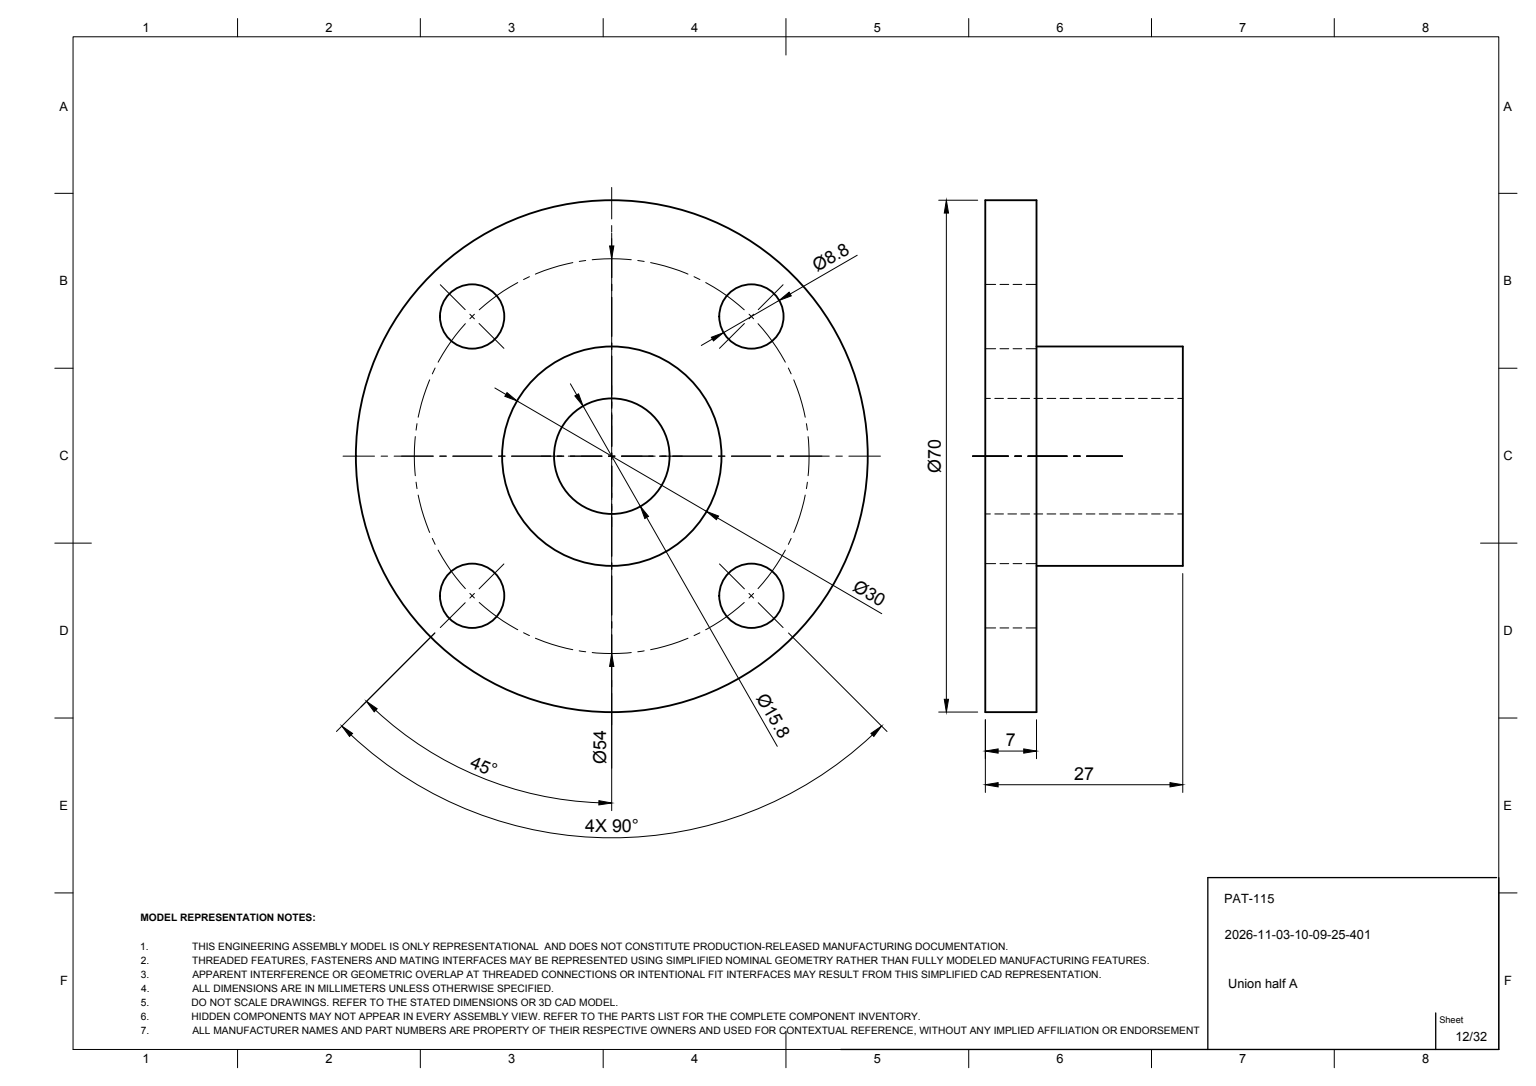
ISO-10303-21;
HEADER;
/* Generated by software containing ST-Developer
 * from STEP Tools, Inc. (www.steptools.com) 
 */

FILE_DESCRIPTION(
/* description */ ('Union bypass pipe loop'),
/* implementation_level */ '2;1');

FILE_NAME(
/* name */ 'Union half A.step',
/* time_stamp */ '2026-10-27T21:00:29-07:00',
/* author */ (''),
/* organization */ (''),
/* preprocessor_version */ 'ST-DEVELOPER v20.2',
/* originating_system */ 'Autodesk Translation Framework v15.17.0.0',
/* authorisation */ '');

FILE_SCHEMA (('AUTOMOTIVE_DESIGN { 1 0 10303 214 3 1 1 }'));
ENDSEC;

DATA;
#10=MECHANICAL_DESIGN_GEOMETRIC_PRESENTATION_REPRESENTATION('',(#466),#10095);
#402=SHAPE_REPRESENTATION_RELATIONSHIP('SRR','None',#10271,#434);
#434=ADVANCED_BREP_SHAPE_REPRESENTATION('',(#496),#10083);
#466=STYLED_ITEM('',(#10514),#496);
#496=MANIFOLD_SOLID_BREP('Body1',#5539);
#599=FACE_BOUND('',#1475,.T.);
#600=FACE_BOUND('',#1476,.T.);
#601=FACE_BOUND('',#1477,.T.);
#602=FACE_BOUND('',#1478,.T.);
#603=FACE_BOUND('',#1479,.T.);
#604=FACE_BOUND('',#1484,.T.);
#605=FACE_BOUND('',#1485,.T.);
#606=FACE_BOUND('',#1486,.T.);
#607=FACE_BOUND('',#1487,.T.);
#608=FACE_BOUND('',#1488,.T.);
#609=FACE_BOUND('',#1490,.T.);
#754=PLANE('',#6388);
#755=PLANE('',#6398);
#756=PLANE('',#6399);
#1050=FACE_OUTER_BOUND('',#1470,.T.);
#1051=FACE_OUTER_BOUND('',#1471,.T.);
#1052=FACE_OUTER_BOUND('',#1472,.T.);
#1053=FACE_OUTER_BOUND('',#1473,.T.);
#1054=FACE_OUTER_BOUND('',#1474,.T.);
#1055=FACE_OUTER_BOUND('',#1480,.T.);
#1056=FACE_OUTER_BOUND('',#1481,.T.);
#1057=FACE_OUTER_BOUND('',#1482,.T.);
#1058=FACE_OUTER_BOUND('',#1483,.T.);
#1059=FACE_OUTER_BOUND('',#1489,.T.);
#1470=EDGE_LOOP('',(#4600,#4601,#4602,#4603));
#1471=EDGE_LOOP('',(#4604,#4605,#4606,#4607));
#1472=EDGE_LOOP('',(#4608,#4609,#4610,#4611));
#1473=EDGE_LOOP('',(#4612,#4613,#4614,#4615));
#1474=EDGE_LOOP('',(#4616));
#1475=EDGE_LOOP('',(#4617));
#1476=EDGE_LOOP('',(#4618));
#1477=EDGE_LOOP('',(#4619));
#1478=EDGE_LOOP('',(#4620));
#1479=EDGE_LOOP('',(#4621));
#1480=EDGE_LOOP('',(#4622,#4623,#4624,#4625));
#1481=EDGE_LOOP('',(#4626,#4627,#4628,#4629));
#1482=EDGE_LOOP('',(#4630,#4631,#4632,#4633));
#1483=EDGE_LOOP('',(#4634));
#1484=EDGE_LOOP('',(#4635));
#1485=EDGE_LOOP('',(#4636));
#1486=EDGE_LOOP('',(#4637));
#1487=EDGE_LOOP('',(#4638));
#1488=EDGE_LOOP('',(#4639));
#1489=EDGE_LOOP('',(#4640));
#1490=EDGE_LOOP('',(#4641));
#1846=LINE('',#9439,#2222);
#1847=LINE('',#9445,#2223);
#1848=LINE('',#9451,#2224);
#1849=LINE('',#9457,#2225);
#1850=LINE('',#9467,#2226);
#1851=LINE('',#9472,#2227);
#1852=LINE('',#9476,#2228);
#2222=VECTOR('',#7788,0.44);
#2223=VECTOR('',#7795,0.44);
#2224=VECTOR('',#7802,0.44);
#2225=VECTOR('',#7809,0.44);
#2226=VECTOR('',#7822,3.5);
#2227=VECTOR('',#7827,0.79);
#2228=VECTOR('',#7832,1.5);
#2555=CIRCLE('',#6377,0.44);
#2556=CIRCLE('',#6378,0.44);
#2557=CIRCLE('',#6380,0.44);
#2558=CIRCLE('',#6381,0.44);
#2559=CIRCLE('',#6383,0.44);
#2560=CIRCLE('',#6384,0.44);
#2561=CIRCLE('',#6386,0.44);
#2562=CIRCLE('',#6387,0.44);
#2563=CIRCLE('',#6389,3.5);
#2564=CIRCLE('',#6390,1.5);
#2565=CIRCLE('',#6392,3.5);
#2566=CIRCLE('',#6394,0.79);
#2567=CIRCLE('',#6395,0.79);
#2568=CIRCLE('',#6397,1.5);
#2912=VERTEX_POINT('',#9436);
#2913=VERTEX_POINT('',#9438);
#2914=VERTEX_POINT('',#9442);
#2915=VERTEX_POINT('',#9444);
#2916=VERTEX_POINT('',#9448);
#2917=VERTEX_POINT('',#9450);
#2918=VERTEX_POINT('',#9454);
#2919=VERTEX_POINT('',#9456);
#2920=VERTEX_POINT('',#9460);
#2921=VERTEX_POINT('',#9462);
#2922=VERTEX_POINT('',#9465);
#2923=VERTEX_POINT('',#9469);
#2924=VERTEX_POINT('',#9471);
#2925=VERTEX_POINT('',#9475);
#3498=EDGE_CURVE('',#2912,#2912,#2555,.T.);
#3499=EDGE_CURVE('',#2912,#2913,#1846,.T.);
#3500=EDGE_CURVE('',#2913,#2913,#2556,.T.);
#3501=EDGE_CURVE('',#2914,#2914,#2557,.T.);
#3502=EDGE_CURVE('',#2914,#2915,#1847,.T.);
#3503=EDGE_CURVE('',#2915,#2915,#2558,.T.);
#3504=EDGE_CURVE('',#2916,#2916,#2559,.T.);
#3505=EDGE_CURVE('',#2916,#2917,#1848,.T.);
#3506=EDGE_CURVE('',#2917,#2917,#2560,.T.);
#3507=EDGE_CURVE('',#2918,#2918,#2561,.T.);
#3508=EDGE_CURVE('',#2918,#2919,#1849,.T.);
#3509=EDGE_CURVE('',#2919,#2919,#2562,.T.);
#3510=EDGE_CURVE('',#2920,#2920,#2563,.T.);
#3511=EDGE_CURVE('',#2921,#2921,#2564,.T.);
#3512=EDGE_CURVE('',#2922,#2922,#2565,.T.);
#3513=EDGE_CURVE('',#2922,#2920,#1850,.T.);
#3514=EDGE_CURVE('',#2923,#2923,#2566,.T.);
#3515=EDGE_CURVE('',#2923,#2924,#1851,.T.);
#3516=EDGE_CURVE('',#2924,#2924,#2567,.T.);
#3517=EDGE_CURVE('',#2921,#2925,#1852,.T.);
#3518=EDGE_CURVE('',#2925,#2925,#2568,.T.);
#4600=ORIENTED_EDGE('',*,*,#3498,.F.);
#4601=ORIENTED_EDGE('',*,*,#3499,.T.);
#4602=ORIENTED_EDGE('',*,*,#3500,.F.);
#4603=ORIENTED_EDGE('',*,*,#3499,.F.);
#4604=ORIENTED_EDGE('',*,*,#3501,.F.);
#4605=ORIENTED_EDGE('',*,*,#3502,.T.);
#4606=ORIENTED_EDGE('',*,*,#3503,.F.);
#4607=ORIENTED_EDGE('',*,*,#3502,.F.);
#4608=ORIENTED_EDGE('',*,*,#3504,.F.);
#4609=ORIENTED_EDGE('',*,*,#3505,.T.);
#4610=ORIENTED_EDGE('',*,*,#3506,.F.);
#4611=ORIENTED_EDGE('',*,*,#3505,.F.);
#4612=ORIENTED_EDGE('',*,*,#3507,.F.);
#4613=ORIENTED_EDGE('',*,*,#3508,.T.);
#4614=ORIENTED_EDGE('',*,*,#3509,.F.);
#4615=ORIENTED_EDGE('',*,*,#3508,.F.);
#4616=ORIENTED_EDGE('',*,*,#3510,.F.);
#4617=ORIENTED_EDGE('',*,*,#3511,.F.);
#4618=ORIENTED_EDGE('',*,*,#3507,.T.);
#4619=ORIENTED_EDGE('',*,*,#3504,.T.);
#4620=ORIENTED_EDGE('',*,*,#3501,.T.);
#4621=ORIENTED_EDGE('',*,*,#3498,.T.);
#4622=ORIENTED_EDGE('',*,*,#3512,.F.);
#4623=ORIENTED_EDGE('',*,*,#3513,.T.);
#4624=ORIENTED_EDGE('',*,*,#3510,.T.);
#4625=ORIENTED_EDGE('',*,*,#3513,.F.);
#4626=ORIENTED_EDGE('',*,*,#3514,.F.);
#4627=ORIENTED_EDGE('',*,*,#3515,.T.);
#4628=ORIENTED_EDGE('',*,*,#3516,.T.);
#4629=ORIENTED_EDGE('',*,*,#3515,.F.);
#4630=ORIENTED_EDGE('',*,*,#3511,.T.);
#4631=ORIENTED_EDGE('',*,*,#3517,.T.);
#4632=ORIENTED_EDGE('',*,*,#3518,.T.);
#4633=ORIENTED_EDGE('',*,*,#3517,.F.);
#4634=ORIENTED_EDGE('',*,*,#3512,.T.);
#4635=ORIENTED_EDGE('',*,*,#3514,.T.);
#4636=ORIENTED_EDGE('',*,*,#3509,.T.);
#4637=ORIENTED_EDGE('',*,*,#3506,.T.);
#4638=ORIENTED_EDGE('',*,*,#3503,.T.);
#4639=ORIENTED_EDGE('',*,*,#3500,.T.);
#4640=ORIENTED_EDGE('',*,*,#3518,.F.);
#4641=ORIENTED_EDGE('',*,*,#3516,.F.);
#5158=CYLINDRICAL_SURFACE('',#6376,0.44);
#5159=CYLINDRICAL_SURFACE('',#6379,0.44);
#5160=CYLINDRICAL_SURFACE('',#6382,0.44);
#5161=CYLINDRICAL_SURFACE('',#6385,0.44);
#5162=CYLINDRICAL_SURFACE('',#6391,3.5);
#5163=CYLINDRICAL_SURFACE('',#6393,0.79);
#5164=CYLINDRICAL_SURFACE('',#6396,1.5);
#5399=ADVANCED_FACE('',(#1050),#5158,.F.);
#5400=ADVANCED_FACE('',(#1051),#5159,.F.);
#5401=ADVANCED_FACE('',(#1052),#5160,.F.);
#5402=ADVANCED_FACE('',(#1053),#5161,.F.);
#5403=ADVANCED_FACE('',(#1054,#599,#600,#601,#602,#603),#754,.F.);
#5404=ADVANCED_FACE('',(#1055),#5162,.T.);
#5405=ADVANCED_FACE('',(#1056),#5163,.F.);
#5406=ADVANCED_FACE('',(#1057),#5164,.T.);
#5407=ADVANCED_FACE('',(#1058,#604,#605,#606,#607,#608),#755,.T.);
#5408=ADVANCED_FACE('',(#1059,#609),#756,.F.);
#5539=CLOSED_SHELL('',(#5399,#5400,#5401,#5402,#5403,#5404,#5405,#5406,
#5407,#5408));
#6375=AXIS2_PLACEMENT_3D('',#9434,#7782,#7783);
#6376=AXIS2_PLACEMENT_3D('',#9435,#7784,#7785);
#6377=AXIS2_PLACEMENT_3D('',#9437,#7786,#7787);
#6378=AXIS2_PLACEMENT_3D('',#9440,#7789,#7790);
#6379=AXIS2_PLACEMENT_3D('',#9441,#7791,#7792);
#6380=AXIS2_PLACEMENT_3D('',#9443,#7793,#7794);
#6381=AXIS2_PLACEMENT_3D('',#9446,#7796,#7797);
#6382=AXIS2_PLACEMENT_3D('',#9447,#7798,#7799);
#6383=AXIS2_PLACEMENT_3D('',#9449,#7800,#7801);
#6384=AXIS2_PLACEMENT_3D('',#9452,#7803,#7804);
#6385=AXIS2_PLACEMENT_3D('',#9453,#7805,#7806);
#6386=AXIS2_PLACEMENT_3D('',#9455,#7807,#7808);
#6387=AXIS2_PLACEMENT_3D('',#9458,#7810,#7811);
#6388=AXIS2_PLACEMENT_3D('',#9459,#7812,#7813);
#6389=AXIS2_PLACEMENT_3D('',#9461,#7814,#7815);
#6390=AXIS2_PLACEMENT_3D('',#9463,#7816,#7817);
#6391=AXIS2_PLACEMENT_3D('',#9464,#7818,#7819);
#6392=AXIS2_PLACEMENT_3D('',#9466,#7820,#7821);
#6393=AXIS2_PLACEMENT_3D('',#9468,#7823,#7824);
#6394=AXIS2_PLACEMENT_3D('',#9470,#7825,#7826);
#6395=AXIS2_PLACEMENT_3D('',#9473,#7828,#7829);
#6396=AXIS2_PLACEMENT_3D('',#9474,#7830,#7831);
#6397=AXIS2_PLACEMENT_3D('',#9477,#7833,#7834);
#6398=AXIS2_PLACEMENT_3D('',#9478,#7835,#7836);
#6399=AXIS2_PLACEMENT_3D('',#9479,#7837,#7838);
#7782=DIRECTION('axis',(0.,0.,1.));
#7783=DIRECTION('refdir',(1.,0.,0.));
#7784=DIRECTION('center_axis',(1.,0.,0.));
#7785=DIRECTION('ref_axis',(0.,0.,-1.));
#7786=DIRECTION('center_axis',(1.,0.,0.));
#7787=DIRECTION('ref_axis',(0.,0.,-1.));
#7788=DIRECTION('',(1.,0.,0.));
#7789=DIRECTION('center_axis',(-1.,0.,0.));
#7790=DIRECTION('ref_axis',(0.,0.,-1.));
#7791=DIRECTION('center_axis',(1.,0.,0.));
#7792=DIRECTION('ref_axis',(0.,0.,-1.));
#7793=DIRECTION('center_axis',(1.,0.,0.));
#7794=DIRECTION('ref_axis',(0.,0.,-1.));
#7795=DIRECTION('',(1.,0.,0.));
#7796=DIRECTION('center_axis',(-1.,0.,0.));
#7797=DIRECTION('ref_axis',(0.,0.,-1.));
#7798=DIRECTION('center_axis',(1.,0.,0.));
#7799=DIRECTION('ref_axis',(0.,0.,-1.));
#7800=DIRECTION('center_axis',(1.,0.,0.));
#7801=DIRECTION('ref_axis',(0.,0.,-1.));
#7802=DIRECTION('',(1.,0.,0.));
#7803=DIRECTION('center_axis',(-1.,0.,0.));
#7804=DIRECTION('ref_axis',(0.,0.,-1.));
#7805=DIRECTION('center_axis',(1.,0.,0.));
#7806=DIRECTION('ref_axis',(0.,0.,-1.));
#7807=DIRECTION('center_axis',(1.,0.,0.));
#7808=DIRECTION('ref_axis',(0.,0.,-1.));
#7809=DIRECTION('',(1.,0.,0.));
#7810=DIRECTION('center_axis',(-1.,0.,0.));
#7811=DIRECTION('ref_axis',(0.,0.,-1.));
#7812=DIRECTION('center_axis',(1.,0.,0.));
#7813=DIRECTION('ref_axis',(0.,0.,-1.));
#7814=DIRECTION('center_axis',(1.,0.,0.));
#7815=DIRECTION('ref_axis',(0.,0.,-1.));
#7816=DIRECTION('center_axis',(-1.,0.,0.));
#7817=DIRECTION('ref_axis',(0.,0.,-1.));
#7818=DIRECTION('center_axis',(1.,0.,0.));
#7819=DIRECTION('ref_axis',(0.,0.,-1.));
#7820=DIRECTION('center_axis',(1.,0.,0.));
#7821=DIRECTION('ref_axis',(0.,0.,-1.));
#7822=DIRECTION('',(-1.,0.,0.));
#7823=DIRECTION('center_axis',(1.,0.,0.));
#7824=DIRECTION('ref_axis',(0.,0.,-1.));
#7825=DIRECTION('center_axis',(-1.,0.,0.));
#7826=DIRECTION('ref_axis',(0.,0.,-1.));
#7827=DIRECTION('',(-1.,0.,0.));
#7828=DIRECTION('center_axis',(-1.,0.,0.));
#7829=DIRECTION('ref_axis',(0.,0.,-1.));
#7830=DIRECTION('center_axis',(1.,0.,0.));
#7831=DIRECTION('ref_axis',(0.,0.,-1.));
#7832=DIRECTION('',(-1.,0.,0.));
#7833=DIRECTION('center_axis',(1.,0.,0.));
#7834=DIRECTION('ref_axis',(0.,0.,-1.));
#7835=DIRECTION('center_axis',(1.,0.,0.));
#7836=DIRECTION('ref_axis',(0.,0.,-1.));
#7837=DIRECTION('center_axis',(1.,0.,0.));
#7838=DIRECTION('ref_axis',(0.,0.,-1.));
#9434=CARTESIAN_POINT('',(0.,0.,0.));
#9435=CARTESIAN_POINT('Origin',(-0.9,-1.90918830920368,4.09081169079632));
#9436=CARTESIAN_POINT('',(-0.8,-1.90918830920368,4.53081169079632));
#9437=CARTESIAN_POINT('Origin',(-0.8,-1.90918830920368,4.09081169079632));
#9438=CARTESIAN_POINT('',(-0.1,-1.90918830920368,4.53081169079632));
#9439=CARTESIAN_POINT('',(-0.9,-1.90918830920368,4.53081169079632));
#9440=CARTESIAN_POINT('Origin',(-0.1,-1.90918830920368,4.09081169079632));
#9441=CARTESIAN_POINT('Origin',(-0.9,-1.90918830920368,7.90918830920368));
#9442=CARTESIAN_POINT('',(-0.8,-1.90918830920368,8.34918830920368));
#9443=CARTESIAN_POINT('Origin',(-0.8,-1.90918830920368,7.90918830920368));
#9444=CARTESIAN_POINT('',(-0.1,-1.90918830920368,8.34918830920368));
#9445=CARTESIAN_POINT('',(-0.9,-1.90918830920368,8.34918830920368));
#9446=CARTESIAN_POINT('Origin',(-0.1,-1.90918830920368,7.90918830920368));
#9447=CARTESIAN_POINT('Origin',(-0.9,1.90918830920368,7.90918830920368));
#9448=CARTESIAN_POINT('',(-0.8,1.90918830920368,8.34918830920368));
#9449=CARTESIAN_POINT('Origin',(-0.8,1.90918830920368,7.90918830920368));
#9450=CARTESIAN_POINT('',(-0.1,1.90918830920368,8.34918830920368));
#9451=CARTESIAN_POINT('',(-0.9,1.90918830920368,8.34918830920368));
#9452=CARTESIAN_POINT('Origin',(-0.1,1.90918830920368,7.90918830920368));
#9453=CARTESIAN_POINT('Origin',(-0.9,1.90918830920368,4.09081169079632));
#9454=CARTESIAN_POINT('',(-0.8,1.90918830920368,4.53081169079632));
#9455=CARTESIAN_POINT('Origin',(-0.8,1.90918830920368,4.09081169079632));
#9456=CARTESIAN_POINT('',(-0.1,1.90918830920368,4.53081169079632));
#9457=CARTESIAN_POINT('',(-0.9,1.90918830920368,4.53081169079632));
#9458=CARTESIAN_POINT('Origin',(-0.1,1.90918830920368,4.09081169079632));
#9459=CARTESIAN_POINT('Origin',(-0.8,0.,6.));
#9460=CARTESIAN_POINT('',(-0.8,-4.28626379701574E-16,9.5));
#9461=CARTESIAN_POINT('Origin',(-0.8,0.,6.));
#9462=CARTESIAN_POINT('',(-0.8,1.83697019872103E-16,7.5));
#9463=CARTESIAN_POINT('Origin',(-0.8,0.,6.));
#9464=CARTESIAN_POINT('Origin',(-0.8,0.,6.));
#9465=CARTESIAN_POINT('',(-0.1,-4.28626379701574E-16,9.5));
#9466=CARTESIAN_POINT('Origin',(-0.1,0.,6.));
#9467=CARTESIAN_POINT('',(-0.8,-4.28626379701574E-16,9.5));
#9468=CARTESIAN_POINT('Origin',(-2.8,0.,6.));
#9469=CARTESIAN_POINT('',(-0.1,-9.67470971326409E-17,6.79));
#9470=CARTESIAN_POINT('Origin',(-0.1,0.,6.));
#9471=CARTESIAN_POINT('',(-2.8,-9.67470971326409E-17,6.79));
#9472=CARTESIAN_POINT('',(-2.8,-9.67470971326409E-17,6.79));
#9473=CARTESIAN_POINT('Origin',(-2.8,0.,6.));
#9474=CARTESIAN_POINT('Origin',(-2.8,0.,6.));
#9475=CARTESIAN_POINT('',(-2.8,-1.83697019872103E-16,7.5));
#9476=CARTESIAN_POINT('',(-2.8,-1.83697019872103E-16,7.5));
#9477=CARTESIAN_POINT('Origin',(-2.8,0.,6.));
#9478=CARTESIAN_POINT('Origin',(-0.1,0.,6.));
#9479=CARTESIAN_POINT('Origin',(-2.8,0.,6.));
#10046=UNCERTAINTY_MEASURE_WITH_UNIT(LENGTH_MEASURE(0.001),#10096,
'DISTANCE_ACCURACY_VALUE',
'Maximum model space distance between geometric entities at asserted c
onnectivities');
#10058=UNCERTAINTY_MEASURE_WITH_UNIT(LENGTH_MEASURE(0.001),#10096,
'DISTANCE_ACCURACY_VALUE',
'Maximum model space distance between geometric entities at asserted c
onnectivities');
#10083=(
GEOMETRIC_REPRESENTATION_CONTEXT(3)
GLOBAL_UNCERTAINTY_ASSIGNED_CONTEXT((#10046))
GLOBAL_UNIT_ASSIGNED_CONTEXT((#10096,#10098,#10099))
REPRESENTATION_CONTEXT('','3D')
);
#10095=(
GEOMETRIC_REPRESENTATION_CONTEXT(3)
GLOBAL_UNCERTAINTY_ASSIGNED_CONTEXT((#10058))
GLOBAL_UNIT_ASSIGNED_CONTEXT((#10096,#10098,#10099))
REPRESENTATION_CONTEXT('','3D')
);
#10096=(
LENGTH_UNIT()
NAMED_UNIT(*)
SI_UNIT(.CENTI.,.METRE.)
);
#10098=(
NAMED_UNIT(*)
PLANE_ANGLE_UNIT()
SI_UNIT($,.RADIAN.)
);
#10099=(
NAMED_UNIT(*)
SI_UNIT($,.STERADIAN.)
SOLID_ANGLE_UNIT()
);
#10124=SHAPE_DEFINITION_REPRESENTATION(#10195,#10271);
#10195=PRODUCT_DEFINITION_SHAPE('',$,#10308);
#10271=SHAPE_REPRESENTATION('',(#6375),#10083);
#10283=PRODUCT_DEFINITION_CONTEXT('part definition',#10393,'design');
#10308=PRODUCT_DEFINITION('Union half A','Union half A',#10344,#10283);
#10344=PRODUCT_DEFINITION_FORMATION('',$,#10419);
#10393=APPLICATION_CONTEXT(
'Core Data for Automotive Mechanical Design Process');
#10394=PRODUCT_CONTEXT('part definition',#10393,'mechanical');
#10419=PRODUCT('Union half A','Union half A','Union half A',(#10394));
#10508=COLOUR_RGB('Off White',0.89,0.88,0.83);
#10509=FILL_AREA_STYLE_COLOUR('',#10508);
#10510=FILL_AREA_STYLE('',(#10509));
#10511=SURFACE_STYLE_FILL_AREA(#10510);
#10512=SURFACE_SIDE_STYLE('',(#10511));
#10513=SURFACE_STYLE_USAGE(.BOTH.,#10512);
#10514=PRESENTATION_STYLE_ASSIGNMENT((#10513));
ENDSEC;
END-ISO-10303-21;
